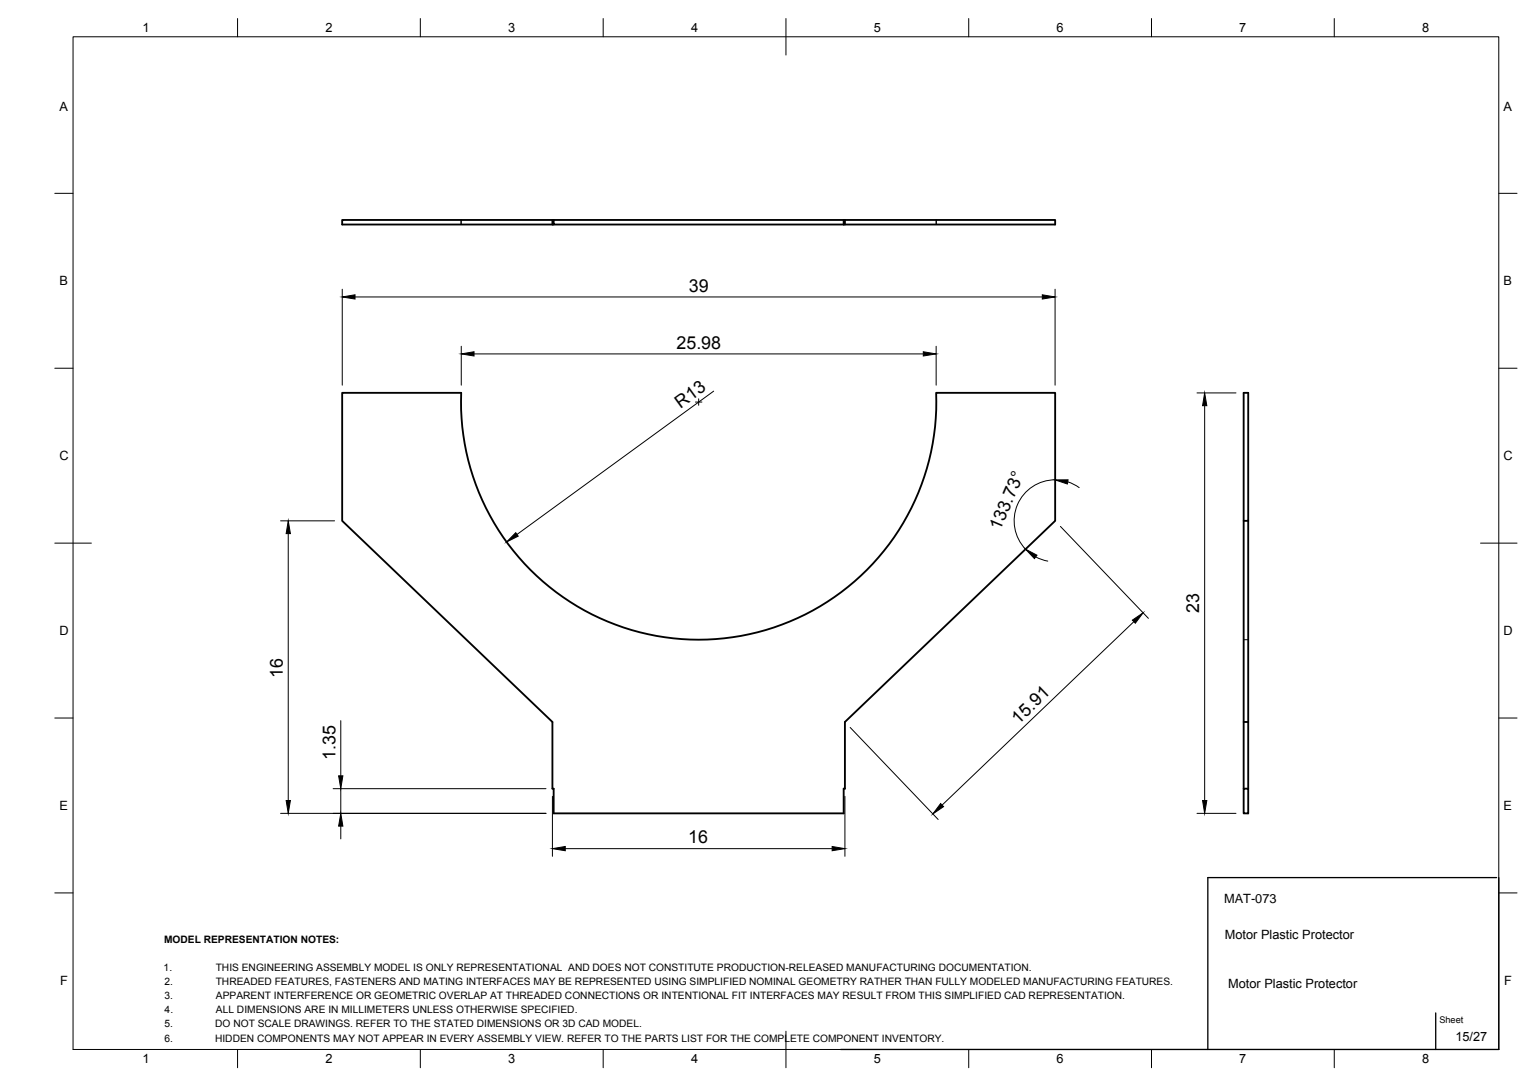
ISO-10303-21;
HEADER;
/* Generated by software containing ST-Developer
 * from STEP Tools, Inc. (www.steptools.com) 
 */

FILE_DESCRIPTION(
/* description */ ('CAx-IF Rec.Pracs.---Representation and Presentation of Product Manufa
cturing Information (PMI)---4.0---2014-10-13'),
/* implementation_level */ '2;1');

FILE_NAME(
/* name */ 'Motor Plastic Protector.step',
/* time_stamp */ '2026-10-24T18:52:33-07:00',
/* author */ (''),
/* organization */ (''),
/* preprocessor_version */ 'ST-DEVELOPER v20.2',
/* originating_system */ 'Autodesk Translation Framework v15.17.0.0',
/* authorisation */ '');

FILE_SCHEMA (('AP242_MANAGED_MODEL_BASED_3D_ENGINEERING_MIM_LF { 1 0 10303 442 2 1 4 }'));
ENDSEC;

DATA;
#10=MECHANICAL_DESIGN_GEOMETRIC_PRESENTATION_REPRESENTATION('',(#428),#34876);
#362=SHAPE_REPRESENTATION_RELATIONSHIP('SRR','None',#34999,#395);
#395=ADVANCED_BREP_SHAPE_REPRESENTATION('',(#461),#34857);
#428=STYLED_ITEM('',(#35160),#461);
#461=MANIFOLD_SOLID_BREP('Motor Plastic Protector',#19568);
#867=PLANE('',#21197);
#868=PLANE('',#21198);
#869=PLANE('',#21199);
#870=PLANE('',#21200);
#871=PLANE('',#21201);
#872=PLANE('',#21202);
#873=PLANE('',#21204);
#874=PLANE('',#21205);
#875=PLANE('',#21206);
#876=PLANE('',#21207);
#877=PLANE('',#21208);
#878=PLANE('',#21211);
#879=PLANE('',#21212);
#880=PLANE('',#21213);
#881=PLANE('',#21214);
#1907=LINE('',#31862,#3506);
#1908=LINE('',#31864,#3507);
#1909=LINE('',#31866,#3508);
#1910=LINE('',#31867,#3509);
#1911=LINE('',#31871,#3510);
#1912=LINE('',#31873,#3511);
#1913=LINE('',#31875,#3512);
#1914=LINE('',#31876,#3513);
#1915=LINE('',#31879,#3514);
#1916=LINE('',#31881,#3515);
#1917=LINE('',#31882,#3516);
#1918=LINE('',#31885,#3517);
#1919=LINE('',#31887,#3518);
#1920=LINE('',#31888,#3519);
#1921=LINE('',#31891,#3520);
#1922=LINE('',#31893,#3521);
#1923=LINE('',#31894,#3522);
#1924=LINE('',#31896,#3523);
#1925=LINE('',#31898,#3524);
#1926=LINE('',#31900,#3525);
#1927=LINE('',#31902,#3526);
#1928=LINE('',#31904,#3527);
#1929=LINE('',#31908,#3528);
#1930=LINE('',#31910,#3529);
#1931=LINE('',#31911,#3530);
#1932=LINE('',#31914,#3531);
#1933=LINE('',#31915,#3532);
#1934=LINE('',#31918,#3533);
#1935=LINE('',#31920,#3534);
#1936=LINE('',#31921,#3535);
#1937=LINE('',#31924,#3536);
#1938=LINE('',#31925,#3537);
#1939=LINE('',#31927,#3538);
#1940=LINE('',#31929,#3539);
#1941=LINE('',#31933,#3540);
#1942=LINE('',#31936,#3541);
#1943=LINE('',#31937,#3542);
#1944=LINE('',#31940,#3543);
#1945=LINE('',#31941,#3544);
#1946=LINE('',#31943,#3545);
#3506=VECTOR('',#25576,0.01);
#3507=VECTOR('',#25577,0.01);
#3508=VECTOR('',#25578,0.01);
#3509=VECTOR('',#25579,0.01);
#3510=VECTOR('',#25582,0.01);
#3511=VECTOR('',#25583,0.01);
#3512=VECTOR('',#25584,0.01);
#3513=VECTOR('',#25585,0.01);
#3514=VECTOR('',#25588,0.01);
#3515=VECTOR('',#25589,0.01);
#3516=VECTOR('',#25590,0.01);
#3517=VECTOR('',#25593,0.01);
#3518=VECTOR('',#25594,0.01);
#3519=VECTOR('',#25595,0.01);
#3520=VECTOR('',#25598,1.);
#3521=VECTOR('',#25599,1.);
#3522=VECTOR('',#25600,1.);
#3523=VECTOR('',#25603,1.);
#3524=VECTOR('',#25604,1.);
#3525=VECTOR('',#25605,1.);
#3526=VECTOR('',#25606,1.);
#3527=VECTOR('',#25607,1.);
#3528=VECTOR('',#25610,1.);
#3529=VECTOR('',#25611,1.);
#3530=VECTOR('',#25612,1.);
#3531=VECTOR('',#25615,1.);
#3532=VECTOR('',#25616,1.);
#3533=VECTOR('',#25619,1.);
#3534=VECTOR('',#25620,1.);
#3535=VECTOR('',#25621,1.);
#3536=VECTOR('',#25624,1.);
#3537=VECTOR('',#25625,1.);
#3538=VECTOR('',#25628,1.);
#3539=VECTOR('',#25631,1.);
#3540=VECTOR('',#25636,1.);
#3541=VECTOR('',#25639,1.);
#3542=VECTOR('',#25640,1.);
#3543=VECTOR('',#25643,1.);
#3544=VECTOR('',#25644,1.);
#3545=VECTOR('',#25647,1.);
#4550=CYLINDRICAL_SURFACE('',#21209,0.013);
#5357=FACE_OUTER_BOUND('',#6458,.T.);
#5358=FACE_OUTER_BOUND('',#6459,.T.);
#5359=FACE_OUTER_BOUND('',#6460,.T.);
#5360=FACE_OUTER_BOUND('',#6461,.T.);
#5361=FACE_OUTER_BOUND('',#6462,.T.);
#5362=FACE_OUTER_BOUND('',#6463,.T.);
#5363=FACE_OUTER_BOUND('',#6464,.T.);
#5364=FACE_OUTER_BOUND('',#6465,.T.);
#5365=FACE_OUTER_BOUND('',#6466,.T.);
#5366=FACE_OUTER_BOUND('',#6467,.T.);
#5367=FACE_OUTER_BOUND('',#6468,.T.);
#5368=FACE_OUTER_BOUND('',#6469,.T.);
#5369=FACE_OUTER_BOUND('',#6470,.T.);
#5370=FACE_OUTER_BOUND('',#6471,.T.);
#5371=FACE_OUTER_BOUND('',#6472,.T.);
#5372=FACE_OUTER_BOUND('',#6473,.T.);
#6458=EDGE_LOOP('',(#15830,#15831,#15832,#15833));
#6459=EDGE_LOOP('',(#15834,#15835,#15836,#15837));
#6460=EDGE_LOOP('',(#15838,#15839,#15840,#15841));
#6461=EDGE_LOOP('',(#15842,#15843,#15844,#15845));
#6462=EDGE_LOOP('',(#15846,#15847,#15848,#15849));
#6463=EDGE_LOOP('',(#15850,#15851,#15852,#15853,#15854,#15855,#15856,#15857,
#15858,#15859,#15860,#15861,#15862,#15863));
#6464=EDGE_LOOP('',(#15864,#15865,#15866,#15867));
#6465=EDGE_LOOP('',(#15868,#15869,#15870,#15871));
#6466=EDGE_LOOP('',(#15872,#15873,#15874,#15875));
#6467=EDGE_LOOP('',(#15876,#15877,#15878,#15879));
#6468=EDGE_LOOP('',(#15880,#15881,#15882,#15883));
#6469=EDGE_LOOP('',(#15884,#15885,#15886,#15887));
#6470=EDGE_LOOP('',(#15888,#15889,#15890,#15891));
#6471=EDGE_LOOP('',(#15892,#15893,#15894,#15895));
#6472=EDGE_LOOP('',(#15896,#15897,#15898,#15899));
#6473=EDGE_LOOP('',(#15900,#15901,#15902,#15903,#15904,#15905,#15906,#15907,
#15908,#15909,#15910,#15911,#15912,#15913));
#7547=CIRCLE('',#21203,0.01300000000001);
#7548=CIRCLE('',#21210,0.01300000000001);
#9073=VERTEX_POINT('',#31860);
#9074=VERTEX_POINT('',#31861);
#9075=VERTEX_POINT('',#31863);
#9076=VERTEX_POINT('',#31865);
#9077=VERTEX_POINT('',#31869);
#9078=VERTEX_POINT('',#31870);
#9079=VERTEX_POINT('',#31872);
#9080=VERTEX_POINT('',#31874);
#9081=VERTEX_POINT('',#31878);
#9082=VERTEX_POINT('',#31880);
#9083=VERTEX_POINT('',#31884);
#9084=VERTEX_POINT('',#31886);
#9085=VERTEX_POINT('',#31890);
#9086=VERTEX_POINT('',#31892);
#9087=VERTEX_POINT('',#31897);
#9088=VERTEX_POINT('',#31899);
#9089=VERTEX_POINT('',#31901);
#9090=VERTEX_POINT('',#31903);
#9091=VERTEX_POINT('',#31905);
#9092=VERTEX_POINT('',#31907);
#9093=VERTEX_POINT('',#31909);
#9094=VERTEX_POINT('',#31913);
#9095=VERTEX_POINT('',#31917);
#9096=VERTEX_POINT('',#31919);
#9097=VERTEX_POINT('',#31923);
#9098=VERTEX_POINT('',#31931);
#9099=VERTEX_POINT('',#31935);
#9100=VERTEX_POINT('',#31939);
#11473=EDGE_CURVE('',#9073,#9074,#1907,.T.);
#11474=EDGE_CURVE('',#9073,#9075,#1908,.T.);
#11475=EDGE_CURVE('',#9076,#9075,#1909,.T.);
#11476=EDGE_CURVE('',#9074,#9076,#1910,.T.);
#11477=EDGE_CURVE('',#9077,#9078,#1911,.T.);
#11478=EDGE_CURVE('',#9077,#9079,#1912,.T.);
#11479=EDGE_CURVE('',#9080,#9079,#1913,.T.);
#11480=EDGE_CURVE('',#9078,#9080,#1914,.T.);
#11481=EDGE_CURVE('',#9081,#9073,#1915,.T.);
#11482=EDGE_CURVE('',#9082,#9081,#1916,.T.);
#11483=EDGE_CURVE('',#9075,#9082,#1917,.T.);
#11484=EDGE_CURVE('',#9083,#9077,#1918,.T.);
#11485=EDGE_CURVE('',#9084,#9083,#1919,.T.);
#11486=EDGE_CURVE('',#9079,#9084,#1920,.T.);
#11487=EDGE_CURVE('',#9076,#9085,#1921,.T.);
#11488=EDGE_CURVE('',#9085,#9086,#1922,.T.);
#11489=EDGE_CURVE('',#9074,#9086,#1923,.T.);
#11490=EDGE_CURVE('',#9082,#9083,#1924,.T.);
#11491=EDGE_CURVE('',#9078,#9087,#1925,.T.);
#11492=EDGE_CURVE('',#9087,#9088,#1926,.T.);
#11493=EDGE_CURVE('',#9088,#9089,#1927,.T.);
#11494=EDGE_CURVE('',#9089,#9090,#1928,.T.);
#11495=EDGE_CURVE('',#9091,#9090,#7547,.T.);
#11496=EDGE_CURVE('',#9092,#9091,#1929,.T.);
#11497=EDGE_CURVE('',#9093,#9092,#1930,.T.);
#11498=EDGE_CURVE('',#9085,#9093,#1931,.T.);
#11499=EDGE_CURVE('',#9080,#9094,#1932,.T.);
#11500=EDGE_CURVE('',#9087,#9094,#1933,.T.);
#11501=EDGE_CURVE('',#9089,#9095,#1934,.T.);
#11502=EDGE_CURVE('',#9095,#9096,#1935,.T.);
#11503=EDGE_CURVE('',#9090,#9096,#1936,.T.);
#11504=EDGE_CURVE('',#9088,#9097,#1937,.T.);
#11505=EDGE_CURVE('',#9097,#9095,#1938,.T.);
#11506=EDGE_CURVE('',#9094,#9097,#1939,.T.);
#11507=EDGE_CURVE('',#9081,#9084,#1940,.T.);
#11508=EDGE_CURVE('',#9098,#9096,#7548,.T.);
#11509=EDGE_CURVE('',#9091,#9098,#1941,.T.);
#11510=EDGE_CURVE('',#9099,#9098,#1942,.T.);
#11511=EDGE_CURVE('',#9092,#9099,#1943,.T.);
#11512=EDGE_CURVE('',#9100,#9099,#1944,.T.);
#11513=EDGE_CURVE('',#9093,#9100,#1945,.T.);
#11514=EDGE_CURVE('',#9086,#9100,#1946,.T.);
#15830=ORIENTED_EDGE('',*,*,#11473,.F.);
#15831=ORIENTED_EDGE('',*,*,#11474,.T.);
#15832=ORIENTED_EDGE('',*,*,#11475,.F.);
#15833=ORIENTED_EDGE('',*,*,#11476,.F.);
#15834=ORIENTED_EDGE('',*,*,#11477,.F.);
#15835=ORIENTED_EDGE('',*,*,#11478,.T.);
#15836=ORIENTED_EDGE('',*,*,#11479,.F.);
#15837=ORIENTED_EDGE('',*,*,#11480,.F.);
#15838=ORIENTED_EDGE('',*,*,#11481,.F.);
#15839=ORIENTED_EDGE('',*,*,#11482,.F.);
#15840=ORIENTED_EDGE('',*,*,#11483,.F.);
#15841=ORIENTED_EDGE('',*,*,#11474,.F.);
#15842=ORIENTED_EDGE('',*,*,#11484,.F.);
#15843=ORIENTED_EDGE('',*,*,#11485,.F.);
#15844=ORIENTED_EDGE('',*,*,#11486,.F.);
#15845=ORIENTED_EDGE('',*,*,#11478,.F.);
#15846=ORIENTED_EDGE('',*,*,#11476,.T.);
#15847=ORIENTED_EDGE('',*,*,#11487,.T.);
#15848=ORIENTED_EDGE('',*,*,#11488,.T.);
#15849=ORIENTED_EDGE('',*,*,#11489,.F.);
#15850=ORIENTED_EDGE('',*,*,#11475,.T.);
#15851=ORIENTED_EDGE('',*,*,#11483,.T.);
#15852=ORIENTED_EDGE('',*,*,#11490,.T.);
#15853=ORIENTED_EDGE('',*,*,#11484,.T.);
#15854=ORIENTED_EDGE('',*,*,#11477,.T.);
#15855=ORIENTED_EDGE('',*,*,#11491,.T.);
#15856=ORIENTED_EDGE('',*,*,#11492,.T.);
#15857=ORIENTED_EDGE('',*,*,#11493,.T.);
#15858=ORIENTED_EDGE('',*,*,#11494,.T.);
#15859=ORIENTED_EDGE('',*,*,#11495,.F.);
#15860=ORIENTED_EDGE('',*,*,#11496,.F.);
#15861=ORIENTED_EDGE('',*,*,#11497,.F.);
#15862=ORIENTED_EDGE('',*,*,#11498,.F.);
#15863=ORIENTED_EDGE('',*,*,#11487,.F.);
#15864=ORIENTED_EDGE('',*,*,#11480,.T.);
#15865=ORIENTED_EDGE('',*,*,#11499,.T.);
#15866=ORIENTED_EDGE('',*,*,#11500,.F.);
#15867=ORIENTED_EDGE('',*,*,#11491,.F.);
#15868=ORIENTED_EDGE('',*,*,#11494,.F.);
#15869=ORIENTED_EDGE('',*,*,#11501,.T.);
#15870=ORIENTED_EDGE('',*,*,#11502,.T.);
#15871=ORIENTED_EDGE('',*,*,#11503,.F.);
#15872=ORIENTED_EDGE('',*,*,#11493,.F.);
#15873=ORIENTED_EDGE('',*,*,#11504,.T.);
#15874=ORIENTED_EDGE('',*,*,#11505,.T.);
#15875=ORIENTED_EDGE('',*,*,#11501,.F.);
#15876=ORIENTED_EDGE('',*,*,#11492,.F.);
#15877=ORIENTED_EDGE('',*,*,#11500,.T.);
#15878=ORIENTED_EDGE('',*,*,#11506,.T.);
#15879=ORIENTED_EDGE('',*,*,#11504,.F.);
#15880=ORIENTED_EDGE('',*,*,#11482,.T.);
#15881=ORIENTED_EDGE('',*,*,#11507,.T.);
#15882=ORIENTED_EDGE('',*,*,#11485,.T.);
#15883=ORIENTED_EDGE('',*,*,#11490,.F.);
#15884=ORIENTED_EDGE('',*,*,#11495,.T.);
#15885=ORIENTED_EDGE('',*,*,#11503,.T.);
#15886=ORIENTED_EDGE('',*,*,#11508,.F.);
#15887=ORIENTED_EDGE('',*,*,#11509,.F.);
#15888=ORIENTED_EDGE('',*,*,#11496,.T.);
#15889=ORIENTED_EDGE('',*,*,#11509,.T.);
#15890=ORIENTED_EDGE('',*,*,#11510,.F.);
#15891=ORIENTED_EDGE('',*,*,#11511,.F.);
#15892=ORIENTED_EDGE('',*,*,#11497,.T.);
#15893=ORIENTED_EDGE('',*,*,#11511,.T.);
#15894=ORIENTED_EDGE('',*,*,#11512,.F.);
#15895=ORIENTED_EDGE('',*,*,#11513,.F.);
#15896=ORIENTED_EDGE('',*,*,#11498,.T.);
#15897=ORIENTED_EDGE('',*,*,#11513,.T.);
#15898=ORIENTED_EDGE('',*,*,#11514,.F.);
#15899=ORIENTED_EDGE('',*,*,#11488,.F.);
#15900=ORIENTED_EDGE('',*,*,#11473,.T.);
#15901=ORIENTED_EDGE('',*,*,#11489,.T.);
#15902=ORIENTED_EDGE('',*,*,#11514,.T.);
#15903=ORIENTED_EDGE('',*,*,#11512,.T.);
#15904=ORIENTED_EDGE('',*,*,#11510,.T.);
#15905=ORIENTED_EDGE('',*,*,#11508,.T.);
#15906=ORIENTED_EDGE('',*,*,#11502,.F.);
#15907=ORIENTED_EDGE('',*,*,#11505,.F.);
#15908=ORIENTED_EDGE('',*,*,#11506,.F.);
#15909=ORIENTED_EDGE('',*,*,#11499,.F.);
#15910=ORIENTED_EDGE('',*,*,#11479,.T.);
#15911=ORIENTED_EDGE('',*,*,#11486,.T.);
#15912=ORIENTED_EDGE('',*,*,#11507,.F.);
#15913=ORIENTED_EDGE('',*,*,#11481,.T.);
#19073=ADVANCED_FACE('',(#5357),#867,.F.);
#19074=ADVANCED_FACE('',(#5358),#868,.F.);
#19075=ADVANCED_FACE('',(#5359),#869,.F.);
#19076=ADVANCED_FACE('',(#5360),#870,.F.);
#19077=ADVANCED_FACE('',(#5361),#871,.T.);
#19078=ADVANCED_FACE('',(#5362),#872,.F.);
#19079=ADVANCED_FACE('',(#5363),#873,.F.);
#19080=ADVANCED_FACE('',(#5364),#874,.F.);
#19081=ADVANCED_FACE('',(#5365),#875,.F.);
#19082=ADVANCED_FACE('',(#5366),#876,.F.);
#19083=ADVANCED_FACE('',(#5367),#877,.T.);
#19084=ADVANCED_FACE('',(#5368),#4550,.F.);
#19085=ADVANCED_FACE('',(#5369),#878,.T.);
#19086=ADVANCED_FACE('',(#5370),#879,.T.);
#19087=ADVANCED_FACE('',(#5371),#880,.T.);
#19088=ADVANCED_FACE('',(#5372),#881,.T.);
#19568=CLOSED_SHELL('',(#19073,#19074,#19075,#19076,#19077,#19078,#19079,
#19080,#19081,#19082,#19083,#19084,#19085,#19086,#19087,#19088));
#21196=AXIS2_PLACEMENT_3D('',#31858,#25572,#25573);
#21197=AXIS2_PLACEMENT_3D('',#31859,#25574,#25575);
#21198=AXIS2_PLACEMENT_3D('',#31868,#25580,#25581);
#21199=AXIS2_PLACEMENT_3D('',#31877,#25586,#25587);
#21200=AXIS2_PLACEMENT_3D('',#31883,#25591,#25592);
#21201=AXIS2_PLACEMENT_3D('',#31889,#25596,#25597);
#21202=AXIS2_PLACEMENT_3D('',#31895,#25601,#25602);
#21203=AXIS2_PLACEMENT_3D('',#31906,#25608,#25609);
#21204=AXIS2_PLACEMENT_3D('',#31912,#25613,#25614);
#21205=AXIS2_PLACEMENT_3D('',#31916,#25617,#25618);
#21206=AXIS2_PLACEMENT_3D('',#31922,#25622,#25623);
#21207=AXIS2_PLACEMENT_3D('',#31926,#25626,#25627);
#21208=AXIS2_PLACEMENT_3D('',#31928,#25629,#25630);
#21209=AXIS2_PLACEMENT_3D('',#31930,#25632,#25633);
#21210=AXIS2_PLACEMENT_3D('',#31932,#25634,#25635);
#21211=AXIS2_PLACEMENT_3D('',#31934,#25637,#25638);
#21212=AXIS2_PLACEMENT_3D('',#31938,#25641,#25642);
#21213=AXIS2_PLACEMENT_3D('',#31942,#25645,#25646);
#21214=AXIS2_PLACEMENT_3D('',#31944,#25648,#25649);
#25572=DIRECTION('axis',(0.,0.,1.));
#25573=DIRECTION('refdir',(1.,0.,0.));
#25574=DIRECTION('center_axis',(-1.,0.,-8.67628499512335E-13));
#25575=DIRECTION('ref_axis',(8.67628499512335E-13,-5.79319727271681E-31,
-1.));
#25576=DIRECTION('',(8.67628499512335E-13,5.22733802929053E-29,-1.));
#25577=DIRECTION('',(0.,-1.,0.));
#25578=DIRECTION('',(-8.67628499512335E-13,-5.22733802929053E-29,1.));
#25579=DIRECTION('',(6.4098735490554E-44,-1.,-7.38780889823027E-32));
#25580=DIRECTION('center_axis',(-1.,0.,-8.67628499512335E-13));
#25581=DIRECTION('ref_axis',(8.67628499512335E-13,-5.79319727271681E-31,
-1.));
#25582=DIRECTION('',(-8.67628499512335E-13,-5.22733802929053E-29,1.));
#25583=DIRECTION('',(0.,1.,0.));
#25584=DIRECTION('',(8.67628499512335E-13,5.22733802929053E-29,-1.));
#25585=DIRECTION('',(-5.24091500843978E-44,1.,6.04050582868765E-32));
#25586=DIRECTION('center_axis',(4.64905891561784E-16,0.,1.));
#25587=DIRECTION('ref_axis',(-1.,-2.80259692864963E-45,4.64905891561784E-16));
#25588=DIRECTION('',(-1.,-6.02124417212377E-17,4.64905891561784E-16));
#25589=DIRECTION('',(-6.02124417212377E-17,1.,2.7993118901524E-32));
#25590=DIRECTION('',(1.,6.02124417212377E-17,-4.64905891561784E-16));
#25591=DIRECTION('center_axis',(-4.64905891561784E-16,0.,-1.));
#25592=DIRECTION('ref_axis',(1.,2.80259692864963E-45,-4.64905891561784E-16));
#25593=DIRECTION('',(-1.,-6.02124417212377E-17,4.64905891561784E-16));
#25594=DIRECTION('',(6.02124417212377E-17,-1.,-2.7993118901524E-32));
#25595=DIRECTION('',(1.,6.02124417212377E-17,-4.64905891561784E-16));
#25596=DIRECTION('center_axis',(7.06303505265682E-16,7.38780889823027E-32,
-1.));
#25597=DIRECTION('ref_axis',(-1.,-6.02124417212377E-17,-7.06303505265682E-16));
#25598=DIRECTION('',(-1.,-6.02124417212377E-17,-7.06303505265682E-16));
#25599=DIRECTION('',(-6.02124417212377E-17,1.,3.1349830333987E-32));
#25600=DIRECTION('',(-1.,-6.02124417212377E-17,-7.06303505265682E-16));
#25601=DIRECTION('center_axis',(-6.02124417212377E-17,1.,3.1349830333987E-32));
#25602=DIRECTION('ref_axis',(-7.06303505265682E-16,-7.38780889823028E-32,
1.));
#25603=DIRECTION('',(9.99517454745522E-13,6.01520366628906E-29,1.));
#25604=DIRECTION('',(-1.,-6.02124417212377E-17,9.99517454745522E-13));
#25605=DIRECTION('',(-0.691222645967388,-4.16202032867111E-17,0.722641857147676));
#25606=DIRECTION('',(-1.,-6.02124417212377E-17,9.99834661323986E-13));
#25607=DIRECTION('',(1.00090892313815E-12,6.02985200330567E-29,-1.));
#25608=DIRECTION('center_axis',(6.02124417212377E-17,-1.,-3.1349830333987E-32));
#25609=DIRECTION('ref_axis',(-7.06303505265682E-16,-7.38780889823028E-32,
1.));
#25610=DIRECTION('',(9.99720074379408E-13,6.01642368857876E-29,1.));
#25611=DIRECTION('',(-1.,-6.02124417212377E-17,-1.00102351008273E-12));
#25612=DIRECTION('',(-0.691222645967387,-4.1620203286711E-17,-0.722641857147678));
#25613=DIRECTION('center_axis',(4.82545253477761E-16,6.04050582868765E-32,
-1.));
#25614=DIRECTION('ref_axis',(-6.02124417212377E-17,1.,3.13498303339869E-32));
#25615=DIRECTION('',(-1.,-6.02124417212377E-17,9.99517454745522E-13));
#25616=DIRECTION('',(-6.02124417212377E-17,1.,3.1349830333987E-32));
#25617=DIRECTION('center_axis',(1.,6.02124417212377E-17,9.08923139152315E-16));
#25618=DIRECTION('ref_axis',(6.02124417212377E-17,-1.,-3.1349830333987E-32));
#25619=DIRECTION('',(-6.02124417212377E-17,1.,3.1349830333987E-32));
#25620=DIRECTION('',(1.00090892313815E-12,6.02985200330567E-29,-1.));
#25621=DIRECTION('',(-6.02124417212377E-17,1.,3.1349830333987E-32));
#25622=DIRECTION('center_axis',(1.6533867501343E-16,4.13052756674997E-32,
-1.));
#25623=DIRECTION('ref_axis',(-6.02124417212377E-17,1.,3.13498303339869E-32));
#25624=DIRECTION('',(-6.02124417212377E-17,1.,3.1349830333987E-32));
#25625=DIRECTION('',(-1.,-6.02124417212377E-17,9.99834661323986E-13));
#25626=DIRECTION('center_axis',(-0.722641857147698,-4.35120307088327E-17,
-0.691222645967365));
#25627=DIRECTION('ref_axis',(-6.02124417212376E-17,1.,9.19638474680743E-32));
#25628=DIRECTION('',(-0.691222645967388,-4.16202032867111E-17,0.722641857147676));
#25629=DIRECTION('center_axis',(1.,6.02124417212377E-17,7.06303505265682E-16));
#25630=DIRECTION('ref_axis',(6.02124417212377E-17,-1.,-3.1349830333987E-32));
#25631=DIRECTION('',(9.99517454745522E-13,6.01520366628906E-29,1.));
#25632=DIRECTION('center_axis',(-6.02124417212377E-17,1.,3.1349830333987E-32));
#25633=DIRECTION('ref_axis',(1.,6.02124417212377E-17,7.6753584522305E-16));
#25634=DIRECTION('center_axis',(6.02124417212377E-17,-1.,-3.1349830333987E-32));
#25635=DIRECTION('ref_axis',(-7.06303505265682E-16,-7.38780889823028E-32,
1.));
#25636=DIRECTION('',(-6.02124417212377E-17,1.,3.1349830333987E-32));
#25637=DIRECTION('center_axis',(-1.,-6.02124417212375E-17,-7.06303505265682E-16));
#25638=DIRECTION('ref_axis',(-7.06303505265682E-16,-4.26377885674554E-16,
1.));
#25639=DIRECTION('',(9.99720074379408E-13,6.01642368857876E-29,1.));
#25640=DIRECTION('',(-6.02124417212377E-17,1.,3.1349830333987E-32));
#25641=DIRECTION('center_axis',(1.02351008373001E-15,9.29778716016794E-32,
-1.));
#25642=DIRECTION('ref_axis',(-1.,-6.02124417212377E-17,-1.02351008373001E-15));
#25643=DIRECTION('',(-1.,-6.02124417212377E-17,-1.00102351008273E-12));
#25644=DIRECTION('',(-6.02124417212377E-17,1.,3.1349830333987E-32));
#25645=DIRECTION('center_axis',(0.7226418571477,4.35120307088328E-17,-0.691222645967364));
#25646=DIRECTION('ref_axis',(-0.691222645967364,-4.16202032867096E-17,-0.7226418571477));
#25647=DIRECTION('',(-0.691222645967387,-4.1620203286711E-17,-0.722641857147678));
#25648=DIRECTION('center_axis',(-6.02124417212377E-17,1.,3.1349830333987E-32));
#25649=DIRECTION('ref_axis',(-7.06303505265682E-16,-7.38780889823028E-32,
1.));
#31858=CARTESIAN_POINT('',(0.,0.,0.));
#31859=CARTESIAN_POINT('Origin',(0.0211500000000181,-0.024,-0.00793218971944487));
#31860=CARTESIAN_POINT('',(0.0211500000000181,-0.03075,-0.00793218971944487));
#31861=CARTESIAN_POINT('',(0.0211500000000182,-0.03074999999999,-0.00800000000000999));
#31862=CARTESIAN_POINT('',(0.0211500000000189,-0.03075,-0.00884109485971803));
#31863=CARTESIAN_POINT('',(0.0211500000000181,-0.031,-0.00793218971944487));
#31864=CARTESIAN_POINT('',(0.0211500000000181,-0.024,-0.00793218971944487));
#31865=CARTESIAN_POINT('',(0.0211500000000182,-0.031,-0.00800000000000999));
#31866=CARTESIAN_POINT('',(0.0211500000000189,-0.031,-0.00884109485971803));
#31867=CARTESIAN_POINT('',(0.0211500000000182,-0.0275,-0.008));
#31868=CARTESIAN_POINT('Origin',(0.02115,-0.024,0.0129631448730622));
#31869=CARTESIAN_POINT('',(0.0211500000000044,-0.031,0.00793218971944469));
#31870=CARTESIAN_POINT('',(0.0211500000000043,-0.031,0.00800000000001137));
#31871=CARTESIAN_POINT('',(0.0211500000000099,-0.031,0.00160657243653548));
#31872=CARTESIAN_POINT('',(0.0211500000000044,-0.03075,0.00793218971944469));
#31873=CARTESIAN_POINT('',(0.0211500000000044,-0.024,0.00793218971944469));
#31874=CARTESIAN_POINT('',(0.0211500000000043,-0.03074999999999,0.00800000000001137));
#31875=CARTESIAN_POINT('',(0.0211500000000099,-0.03075,0.00160657243653548));
#31876=CARTESIAN_POINT('',(0.0211500000000043,-0.0275,0.008));
#31877=CARTESIAN_POINT('Origin',(0.02715,-0.024,-0.00793218971944484));
#31878=CARTESIAN_POINT('',(0.022500000000002,-0.03074999999999,-0.00793218971944484));
#31879=CARTESIAN_POINT('',(0.019075,-0.03075,-0.00793218971944484));
#31880=CARTESIAN_POINT('',(0.022500000000002,-0.031,-0.00793218971944484));
#31881=CARTESIAN_POINT('',(0.0225,-0.0275,-0.00793218971944484));
#31882=CARTESIAN_POINT('',(0.019075,-0.031,-0.00793218971944484));
#31883=CARTESIAN_POINT('Origin',(0.0211500000000044,-0.024,0.00793218971944473));
#31884=CARTESIAN_POINT('',(0.0225000000000178,-0.031,0.00793218971944473));
#31885=CARTESIAN_POINT('',(0.0160750000000022,-0.031,0.00793218971944473));
#31886=CARTESIAN_POINT('',(0.0225000000000178,-0.03074999999999,0.00793218971944473));
#31887=CARTESIAN_POINT('',(0.0225,-0.0275,0.00793218971944473));
#31888=CARTESIAN_POINT('',(0.0160750000000022,-0.03075,0.00793218971944473));
#31889=CARTESIAN_POINT('Origin',(0.0225,-0.031,-0.008));
#31890=CARTESIAN_POINT('',(0.0175,-0.031,-0.008));
#31891=CARTESIAN_POINT('',(0.0225000000000099,-0.031,-0.00800000000000999));
#31892=CARTESIAN_POINT('',(0.0175,-0.03075,-0.008));
#31893=CARTESIAN_POINT('',(0.01750000000001,-0.031,-0.00800000000000999));
#31894=CARTESIAN_POINT('',(0.0225000000000099,-0.03074999999999,-0.00800000000000999));
#31895=CARTESIAN_POINT('Origin',(0.011,-0.031,-0.00975));
#31896=CARTESIAN_POINT('',(0.0225000000000099,-0.031,-9.98512365149887E-15));
#31897=CARTESIAN_POINT('',(0.0175,-0.031,0.008));
#31898=CARTESIAN_POINT('',(0.0225000000000099,-0.031,0.00800000000001002));
#31899=CARTESIAN_POINT('',(0.0065,-0.031,0.0195));
#31900=CARTESIAN_POINT('',(0.01750000000001,-0.031,0.00800000000001001));
#31901=CARTESIAN_POINT('',(-0.000500000000000057,-0.031,0.0195));
#31902=CARTESIAN_POINT('',(0.00650000000000994,-0.031,0.01950000000001));
#31903=CARTESIAN_POINT('',(-0.000500000000000053,-0.031,0.0129903810567666));
#31904=CARTESIAN_POINT('',(-0.000500000000010059,-0.031,0.01950000000001));
#31905=CARTESIAN_POINT('',(-0.000500000000000034,-0.031,-0.0129903810567666));
#31906=CARTESIAN_POINT('Origin',(-4.35057343591877E-17,-0.031,8.02542624668979E-33));
#31907=CARTESIAN_POINT('',(-0.000500000000000036,-0.031,-0.0195));
#31908=CARTESIAN_POINT('',(-0.000500000000010036,-0.031,-0.01950000000001));
#31909=CARTESIAN_POINT('',(0.0065,-0.031,-0.0195));
#31910=CARTESIAN_POINT('',(0.00650000000000996,-0.031,-0.01950000000001));
#31911=CARTESIAN_POINT('',(0.01750000000001,-0.031,-0.00800000000000999));
#31912=CARTESIAN_POINT('Origin',(0.0225,-0.031,0.008));
#31913=CARTESIAN_POINT('',(0.0175,-0.03075,0.008));
#31914=CARTESIAN_POINT('',(0.0225000000000099,-0.03074999999999,0.00800000000001002));
#31915=CARTESIAN_POINT('',(0.01750000000001,-0.031,0.00800000000001001));
#31916=CARTESIAN_POINT('Origin',(-0.000500000000000057,-0.031,0.0195));
#31917=CARTESIAN_POINT('',(-0.000500000000000057,-0.03075,0.0195));
#31918=CARTESIAN_POINT('',(-0.000500000000010059,-0.031,0.01950000000001));
#31919=CARTESIAN_POINT('',(-0.000500000000000053,-0.03075,0.0129903810567666));
#31920=CARTESIAN_POINT('',(-0.000500000000010059,-0.03074999999999,0.01950000000001));
#31921=CARTESIAN_POINT('',(-0.000500000000010053,-0.031,0.0129903810567766));
#31922=CARTESIAN_POINT('Origin',(0.0065,-0.031,0.0195));
#31923=CARTESIAN_POINT('',(0.0065,-0.03075,0.0195));
#31924=CARTESIAN_POINT('',(0.00650000000000994,-0.031,0.01950000000001));
#31925=CARTESIAN_POINT('',(0.00650000000000994,-0.03074999999999,0.01950000000001));
#31926=CARTESIAN_POINT('Origin',(0.0175,-0.031,0.008));
#31927=CARTESIAN_POINT('',(0.01750000000001,-0.03074999999999,0.00800000000001001));
#31928=CARTESIAN_POINT('Origin',(0.0225,-0.031,1.48289771724852E-17));
#31929=CARTESIAN_POINT('',(0.0225000000000099,-0.03074999999999,-9.98512365149887E-15));
#31930=CARTESIAN_POINT('Origin',(-4.35057343591877E-17,-0.031,8.02542624668979E-33));
#31931=CARTESIAN_POINT('',(-0.000500000000000034,-0.03075,-0.0129903810567666));
#31932=CARTESIAN_POINT('Origin',(-4.35207874696186E-17,-0.03074999999999,
8.0332637042736E-33));
#31933=CARTESIAN_POINT('',(-0.000500000000010037,-0.031,-0.0129903810567766));
#31934=CARTESIAN_POINT('Origin',(-0.000500000000000036,-0.031,-0.0195));
#31935=CARTESIAN_POINT('',(-0.000500000000000037,-0.03075,-0.0195));
#31936=CARTESIAN_POINT('',(-0.000500000000010036,-0.03074999999999,-0.01950000000001));
#31937=CARTESIAN_POINT('',(-0.000500000000010036,-0.031,-0.01950000000001));
#31938=CARTESIAN_POINT('Origin',(0.0065,-0.031,-0.0195));
#31939=CARTESIAN_POINT('',(0.0065,-0.03075,-0.0195));
#31940=CARTESIAN_POINT('',(0.00650000000000996,-0.03074999999999,-0.01950000000001));
#31941=CARTESIAN_POINT('',(0.00650000000000996,-0.031,-0.01950000000001));
#31942=CARTESIAN_POINT('Origin',(0.0175,-0.031,-0.008));
#31943=CARTESIAN_POINT('',(0.01750000000001,-0.03074999999999,-0.00800000000000999));
#31944=CARTESIAN_POINT('Origin',(0.011,-0.03075,-0.00975));
#34822=UNCERTAINTY_MEASURE_WITH_UNIT(LENGTH_MEASURE(1.E-5),#34877,
'DISTANCE_ACCURACY_VALUE',
'Maximum model space distance between geometric entities at asserted c
onnectivities');
#34841=UNCERTAINTY_MEASURE_WITH_UNIT(LENGTH_MEASURE(1.E-5),#34877,
'DISTANCE_ACCURACY_VALUE',
'Maximum model space distance between geometric entities at asserted c
onnectivities');
#34857=(
GEOMETRIC_REPRESENTATION_CONTEXT(3)
GLOBAL_UNCERTAINTY_ASSIGNED_CONTEXT((#34822))
GLOBAL_UNIT_ASSIGNED_CONTEXT((#34877,#34878,#34879))
REPRESENTATION_CONTEXT('','3D')
);
#34876=(
GEOMETRIC_REPRESENTATION_CONTEXT(3)
GLOBAL_UNCERTAINTY_ASSIGNED_CONTEXT((#34841))
GLOBAL_UNIT_ASSIGNED_CONTEXT((#34877,#34878,#34879))
REPRESENTATION_CONTEXT('','3D')
);
#34877=(
LENGTH_UNIT()
NAMED_UNIT(*)
SI_UNIT($,.METRE.)
);
#34878=(
NAMED_UNIT(*)
PLANE_ANGLE_UNIT()
SI_UNIT($,.RADIAN.)
);
#34879=(
NAMED_UNIT(*)
SI_UNIT($,.STERADIAN.)
SOLID_ANGLE_UNIT()
);
#34895=SHAPE_DEFINITION_REPRESENTATION(#34929,#34999);
#34929=PRODUCT_DEFINITION_SHAPE('',$,#35034);
#34999=SHAPE_REPRESENTATION('',(#21196),#34857);
#35018=PRODUCT_DEFINITION_CONTEXT('part definition',#35122,'design');
#35034=PRODUCT_DEFINITION('Motor Plastic Protector',
'Motor Plastic Protector',#35068,#35018);
#35068=PRODUCT_DEFINITION_FORMATION('',$,#35139);
#35122=APPLICATION_CONTEXT('Managed model based 3d engineering');
#35123=PRODUCT_CONTEXT('part definition',#35122,'mechanical');
#35139=PRODUCT('Motor Plastic Protector','Motor Plastic Protector',
'LEGAL AND USAGE DISCLAIMER: this Data/Model is provided \X2\201C\X0\A
S IS\X2\201D\X0\ for informational and representational only. It is a 
geometric approximation and is NOT engineered, certified, or guarantee
d for dimensional accuracy, exact tolerances, or production-level prec
ision. Vendor disclaims all implied warranties including fitness for a
 particular purpose. DO NOT USE FOR DIRECT PHYSICAL MANUFACTURING, AUT
OMATED PRODUCTION, OR SAFETY-CRITICAL SYSTEMS without independent engi
neering verification and resolution of any design discrepancies.',(#35123));
#35160=PRESENTATION_STYLE_ASSIGNMENT((#35169));
#35169=SURFACE_STYLE_USAGE(.BOTH.,#35178);
#35178=SURFACE_SIDE_STYLE('',(#35187));
#35187=SURFACE_STYLE_FILL_AREA(#35196);
#35196=FILL_AREA_STYLE('Plastic - Glossy (Black)',(#35205));
#35205=FILL_AREA_STYLE_COLOUR('Plastic - Glossy (Black)',#35214);
#35214=COLOUR_RGB('Plastic - Glossy (Black)',0.0980392156862745,0.0980392156862745,
0.0980392156862745);
ENDSEC;
END-ISO-10303-21;
